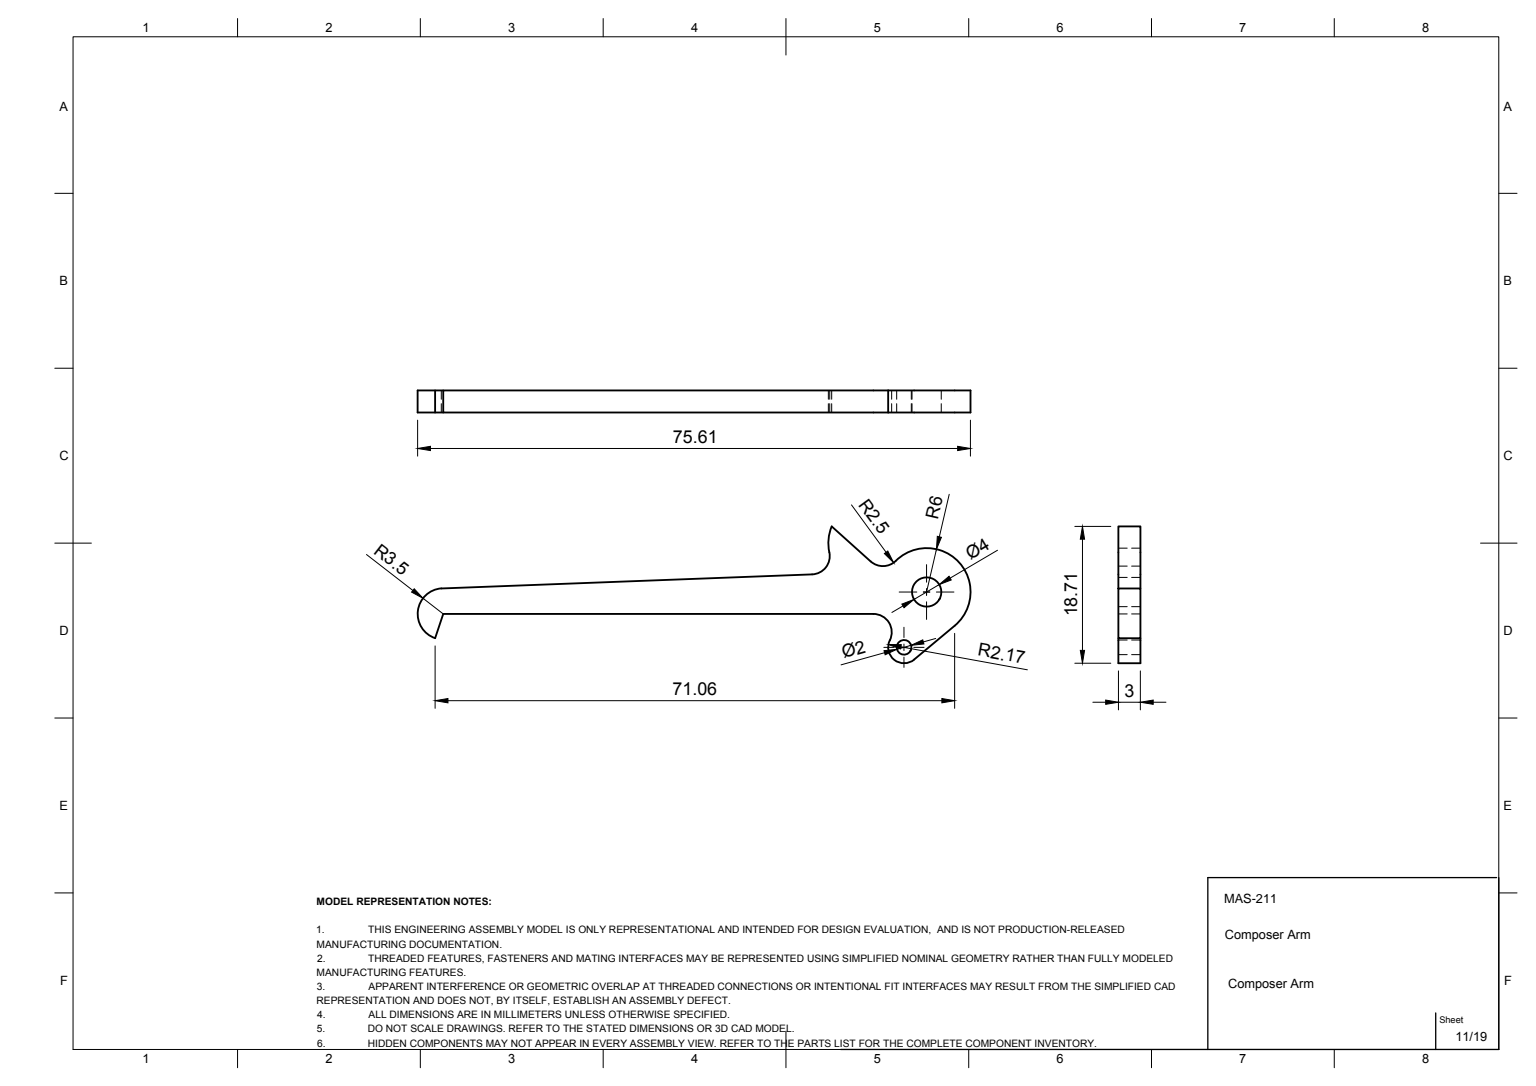
ISO-10303-21;
HEADER;
FILE_DESCRIPTION(
 (''),
 '2;1');
FILE_NAME ( 'Composer Arm.step', '2026-10-05T20:07:59+06:00', ( '' ), ( '' ), 'STEP AP214', 'Unspecified', '' );
FILE_SCHEMA (('AUTOMOTIVE_DESIGN { 1 0 10303 214 3 1 1 }'));
ENDSEC;
DATA;
#10=MECHANICAL_DESIGN_GEOMETRIC_PRESENTATION_REPRESENTATION('',(#328),#196741);
#328=STYLED_ITEM('',(#196765),#347) ;
#347=MANIFOLD_SOLID_BREP('Composer Arm',#8724) ;
#391=PLANE('',#8943) ;
#392=PLANE('',#8950) ;
#393=PLANE('',#8951) ;
#394=PLANE('',#8955) ;
#395=PLANE('',#8962) ;
#396=PLANE('',#8966) ;
#397=PLANE('',#8969) ;
#586=FACE_BOUND('',#1532,.T.) ;
#587=FACE_BOUND('',#1533,.T.) ;
#588=FACE_BOUND('',#1535,.T.) ;
#589=FACE_BOUND('',#1536,.T.) ;
#689=CIRCLE('',#8941,6.00000000000002) ;
#690=CIRCLE('',#8942,6.00000000000002) ;
#691=CIRCLE('',#8945,2.1716132700891) ;
#692=CIRCLE('',#8946,2.1716132700891) ;
#693=CIRCLE('',#8948,2.50000000000001) ;
#694=CIRCLE('',#8949,2.50000000000001) ;
#695=CIRCLE('',#8953,3.49999999999995) ;
#696=CIRCLE('',#8954,3.49999999999995) ;
#697=CIRCLE('',#8957,2.50000000000018) ;
#698=CIRCLE('',#8958,2.50000000000018) ;
#699=CIRCLE('',#8960,5.99999999999934) ;
#700=CIRCLE('',#8961,5.99999999999934) ;
#701=CIRCLE('',#8964,2.49999999999992) ;
#702=CIRCLE('',#8965,2.49999999999992) ;
#703=CIRCLE('',#8967,0.999999999999994) ;
#704=CIRCLE('',#8968,2.00000000000002) ;
#705=CIRCLE('',#8970,0.999999999999994) ;
#706=CIRCLE('',#8971,2.00000000000002) ;
#1014=FACE_OUTER_BOUND('',#1519,.T.) ;
#1015=FACE_OUTER_BOUND('',#1520,.T.) ;
#1016=FACE_OUTER_BOUND('',#1521,.T.) ;
#1017=FACE_OUTER_BOUND('',#1522,.T.) ;
#1018=FACE_OUTER_BOUND('',#1523,.T.) ;
#1019=FACE_OUTER_BOUND('',#1524,.T.) ;
#1020=FACE_OUTER_BOUND('',#1525,.T.) ;
#1021=FACE_OUTER_BOUND('',#1526,.T.) ;
#1022=FACE_OUTER_BOUND('',#1527,.T.) ;
#1023=FACE_OUTER_BOUND('',#1528,.T.) ;
#1024=FACE_OUTER_BOUND('',#1529,.T.) ;
#1025=FACE_OUTER_BOUND('',#1530,.T.) ;
#1026=FACE_OUTER_BOUND('',#1531,.T.) ;
#1027=FACE_OUTER_BOUND('',#1534,.T.) ;
#1028=FACE_OUTER_BOUND('',#1537,.T.) ;
#1029=FACE_OUTER_BOUND('',#1538,.T.) ;
#1519=EDGE_LOOP('',(#6364,#6365,#6366,#6367)) ;
#1520=EDGE_LOOP('',(#6368,#6369,#6370,#6371)) ;
#1521=EDGE_LOOP('',(#6372,#6373,#6374,#6375)) ;
#1522=EDGE_LOOP('',(#6376,#6377,#6378,#6379)) ;
#1523=EDGE_LOOP('',(#6380,#6381,#6382,#6383)) ;
#1524=EDGE_LOOP('',(#6384,#6385,#6386,#6387)) ;
#1525=EDGE_LOOP('',(#6388,#6389,#6390,#6391)) ;
#1526=EDGE_LOOP('',(#6392,#6393,#6394,#6395)) ;
#1527=EDGE_LOOP('',(#6396,#6397,#6398,#6399)) ;
#1528=EDGE_LOOP('',(#6400,#6401,#6402,#6403)) ;
#1529=EDGE_LOOP('',(#6404,#6405,#6406,#6407)) ;
#1530=EDGE_LOOP('',(#6408,#6409,#6410,#6411)) ;
#1531=EDGE_LOOP('',(#6412,#6413,#6414,#6415,#6416,#6417,#6418,#6419,#6420,
#6421,#6422,#6423)) ;
#1532=EDGE_LOOP('',(#6424)) ;
#1533=EDGE_LOOP('',(#6425)) ;
#1534=EDGE_LOOP('',(#6426,#6427,#6428,#6429,#6430,#6431,#6432,#6433,#6434,
#6435,#6436,#6437)) ;
#1535=EDGE_LOOP('',(#6438)) ;
#1536=EDGE_LOOP('',(#6439)) ;
#1537=EDGE_LOOP('',(#6440,#6441,#6442,#6443)) ;
#1538=EDGE_LOOP('',(#6444,#6445,#6446,#6447)) ;
#2010=LINE('',#113918,#2713) ;
#2011=LINE('',#113921,#2714) ;
#2012=LINE('',#113924,#2715) ;
#2013=LINE('',#113926,#2716) ;
#2014=LINE('',#113927,#2717) ;
#2015=LINE('',#113932,#2718) ;
#2016=LINE('',#113938,#2719) ;
#2017=LINE('',#113942,#2720) ;
#2018=LINE('',#113944,#2721) ;
#2019=LINE('',#113945,#2722) ;
#2020=LINE('',#113948,#2723) ;
#2021=LINE('',#113950,#2724) ;
#2022=LINE('',#113951,#2725) ;
#2023=LINE('',#113956,#2726) ;
#2024=LINE('',#113960,#2727) ;
#2025=LINE('',#113962,#2728) ;
#2026=LINE('',#113963,#2729) ;
#2027=LINE('',#113968,#2730) ;
#2028=LINE('',#113974,#2731) ;
#2029=LINE('',#113978,#2732) ;
#2030=LINE('',#113980,#2733) ;
#2031=LINE('',#113981,#2734) ;
#2032=LINE('',#113996,#2735) ;
#2033=LINE('',#113998,#2736) ;
#2713=VECTOR('',#9994,10.) ;
#2714=VECTOR('',#9997,10.) ;
#2715=VECTOR('',#10000,10.) ;
#2716=VECTOR('',#10001,10.) ;
#2717=VECTOR('',#10002,10.) ;
#2718=VECTOR('',#10007,10.) ;
#2719=VECTOR('',#10014,10.) ;
#2720=VECTOR('',#10019,10.) ;
#2721=VECTOR('',#10020,10.) ;
#2722=VECTOR('',#10021,10.) ;
#2723=VECTOR('',#10024,10.) ;
#2724=VECTOR('',#10025,10.) ;
#2725=VECTOR('',#10026,10.) ;
#2726=VECTOR('',#10031,10.) ;
#2727=VECTOR('',#10036,10.) ;
#2728=VECTOR('',#10037,10.) ;
#2729=VECTOR('',#10038,10.) ;
#2730=VECTOR('',#10043,10.) ;
#2731=VECTOR('',#10050,10.) ;
#2732=VECTOR('',#10055,10.) ;
#2733=VECTOR('',#10056,10.) ;
#2734=VECTOR('',#10057,10.) ;
#2735=VECTOR('',#10078,1.00000000000007) ;
#2736=VECTOR('',#10081,2.00000000000001) ;
#3708=VERTEX_POINT('',#113914) ;
#3709=VERTEX_POINT('',#113915) ;
#3710=VERTEX_POINT('',#113917) ;
#3711=VERTEX_POINT('',#113919) ;
#3712=VERTEX_POINT('',#113923) ;
#3713=VERTEX_POINT('',#113925) ;
#3714=VERTEX_POINT('',#113929) ;
#3715=VERTEX_POINT('',#113931) ;
#3716=VERTEX_POINT('',#113935) ;
#3717=VERTEX_POINT('',#113937) ;
#3718=VERTEX_POINT('',#113941) ;
#3719=VERTEX_POINT('',#113943) ;
#3720=VERTEX_POINT('',#113947) ;
#3721=VERTEX_POINT('',#113949) ;
#3722=VERTEX_POINT('',#113953) ;
#3723=VERTEX_POINT('',#113955) ;
#3724=VERTEX_POINT('',#113959) ;
#3725=VERTEX_POINT('',#113961) ;
#3726=VERTEX_POINT('',#113965) ;
#3727=VERTEX_POINT('',#113967) ;
#3728=VERTEX_POINT('',#113971) ;
#3729=VERTEX_POINT('',#113973) ;
#3730=VERTEX_POINT('',#113977) ;
#3731=VERTEX_POINT('',#113979) ;
#3732=VERTEX_POINT('',#113986) ;
#3733=VERTEX_POINT('',#113988) ;
#3734=VERTEX_POINT('',#113991) ;
#3735=VERTEX_POINT('',#113993) ;
#4690=EDGE_CURVE('',#3708,#3709,#689,.T.) ;
#4691=EDGE_CURVE('',#3709,#3710,#2010,.T.) ;
#4692=EDGE_CURVE('',#3711,#3710,#690,.T.) ;
#4693=EDGE_CURVE('',#3708,#3711,#2011,.T.) ;
#4694=EDGE_CURVE('',#3709,#3712,#2012,.T.) ;
#4695=EDGE_CURVE('',#3712,#3713,#2013,.T.) ;
#4696=EDGE_CURVE('',#3710,#3713,#2014,.T.) ;
#4697=EDGE_CURVE('',#3712,#3714,#691,.T.) ;
#4698=EDGE_CURVE('',#3714,#3715,#2015,.T.) ;
#4699=EDGE_CURVE('',#3713,#3715,#692,.T.) ;
#4700=EDGE_CURVE('',#3714,#3716,#693,.T.) ;
#4701=EDGE_CURVE('',#3716,#3717,#2016,.T.) ;
#4702=EDGE_CURVE('',#3715,#3717,#694,.T.) ;
#4703=EDGE_CURVE('',#3716,#3718,#2017,.T.) ;
#4704=EDGE_CURVE('',#3718,#3719,#2018,.T.) ;
#4705=EDGE_CURVE('',#3717,#3719,#2019,.T.) ;
#4706=EDGE_CURVE('',#3718,#3720,#2020,.T.) ;
#4707=EDGE_CURVE('',#3720,#3721,#2021,.T.) ;
#4708=EDGE_CURVE('',#3719,#3721,#2022,.T.) ;
#4709=EDGE_CURVE('',#3720,#3722,#695,.T.) ;
#4710=EDGE_CURVE('',#3722,#3723,#2023,.T.) ;
#4711=EDGE_CURVE('',#3721,#3723,#696,.T.) ;
#4712=EDGE_CURVE('',#3722,#3724,#2024,.T.) ;
#4713=EDGE_CURVE('',#3724,#3725,#2025,.T.) ;
#4714=EDGE_CURVE('',#3723,#3725,#2026,.T.) ;
#4715=EDGE_CURVE('',#3724,#3726,#697,.T.) ;
#4716=EDGE_CURVE('',#3726,#3727,#2027,.T.) ;
#4717=EDGE_CURVE('',#3725,#3727,#698,.T.) ;
#4718=EDGE_CURVE('',#3726,#3728,#699,.T.) ;
#4719=EDGE_CURVE('',#3728,#3729,#2028,.T.) ;
#4720=EDGE_CURVE('',#3727,#3729,#700,.T.) ;
#4721=EDGE_CURVE('',#3728,#3730,#2029,.T.) ;
#4722=EDGE_CURVE('',#3730,#3731,#2030,.T.) ;
#4723=EDGE_CURVE('',#3729,#3731,#2031,.T.) ;
#4724=EDGE_CURVE('',#3730,#3708,#701,.T.) ;
#4725=EDGE_CURVE('',#3731,#3711,#702,.T.) ;
#4726=EDGE_CURVE('',#3732,#3732,#703,.T.) ;
#4727=EDGE_CURVE('',#3733,#3733,#704,.T.) ;
#4728=EDGE_CURVE('',#3734,#3734,#705,.T.) ;
#4729=EDGE_CURVE('',#3735,#3735,#706,.T.) ;
#4730=EDGE_CURVE('',#3734,#3732,#2032,.T.) ;
#4731=EDGE_CURVE('',#3733,#3735,#2033,.T.) ;
#6364=ORIENTED_EDGE('',*,*,#4690,.T.) ;
#6365=ORIENTED_EDGE('',*,*,#4691,.T.) ;
#6366=ORIENTED_EDGE('',*,*,#4692,.F.) ;
#6367=ORIENTED_EDGE('',*,*,#4693,.F.) ;
#6368=ORIENTED_EDGE('',*,*,#4694,.T.) ;
#6369=ORIENTED_EDGE('',*,*,#4695,.T.) ;
#6370=ORIENTED_EDGE('',*,*,#4696,.F.) ;
#6371=ORIENTED_EDGE('',*,*,#4691,.F.) ;
#6372=ORIENTED_EDGE('',*,*,#4697,.T.) ;
#6373=ORIENTED_EDGE('',*,*,#4698,.T.) ;
#6374=ORIENTED_EDGE('',*,*,#4699,.F.) ;
#6375=ORIENTED_EDGE('',*,*,#4695,.F.) ;
#6376=ORIENTED_EDGE('',*,*,#4700,.T.) ;
#6377=ORIENTED_EDGE('',*,*,#4701,.T.) ;
#6378=ORIENTED_EDGE('',*,*,#4702,.F.) ;
#6379=ORIENTED_EDGE('',*,*,#4698,.F.) ;
#6380=ORIENTED_EDGE('',*,*,#4703,.T.) ;
#6381=ORIENTED_EDGE('',*,*,#4704,.T.) ;
#6382=ORIENTED_EDGE('',*,*,#4705,.F.) ;
#6383=ORIENTED_EDGE('',*,*,#4701,.F.) ;
#6384=ORIENTED_EDGE('',*,*,#4706,.T.) ;
#6385=ORIENTED_EDGE('',*,*,#4707,.T.) ;
#6386=ORIENTED_EDGE('',*,*,#4708,.F.) ;
#6387=ORIENTED_EDGE('',*,*,#4704,.F.) ;
#6388=ORIENTED_EDGE('',*,*,#4709,.T.) ;
#6389=ORIENTED_EDGE('',*,*,#4710,.T.) ;
#6390=ORIENTED_EDGE('',*,*,#4711,.F.) ;
#6391=ORIENTED_EDGE('',*,*,#4707,.F.) ;
#6392=ORIENTED_EDGE('',*,*,#4712,.T.) ;
#6393=ORIENTED_EDGE('',*,*,#4713,.T.) ;
#6394=ORIENTED_EDGE('',*,*,#4714,.F.) ;
#6395=ORIENTED_EDGE('',*,*,#4710,.F.) ;
#6396=ORIENTED_EDGE('',*,*,#4715,.T.) ;
#6397=ORIENTED_EDGE('',*,*,#4716,.T.) ;
#6398=ORIENTED_EDGE('',*,*,#4717,.F.) ;
#6399=ORIENTED_EDGE('',*,*,#4713,.F.) ;
#6400=ORIENTED_EDGE('',*,*,#4718,.T.) ;
#6401=ORIENTED_EDGE('',*,*,#4719,.T.) ;
#6402=ORIENTED_EDGE('',*,*,#4720,.F.) ;
#6403=ORIENTED_EDGE('',*,*,#4716,.F.) ;
#6404=ORIENTED_EDGE('',*,*,#4721,.T.) ;
#6405=ORIENTED_EDGE('',*,*,#4722,.T.) ;
#6406=ORIENTED_EDGE('',*,*,#4723,.F.) ;
#6407=ORIENTED_EDGE('',*,*,#4719,.F.) ;
#6408=ORIENTED_EDGE('',*,*,#4724,.T.) ;
#6409=ORIENTED_EDGE('',*,*,#4693,.T.) ;
#6410=ORIENTED_EDGE('',*,*,#4725,.F.) ;
#6411=ORIENTED_EDGE('',*,*,#4722,.F.) ;
#6412=ORIENTED_EDGE('',*,*,#4724,.F.) ;
#6413=ORIENTED_EDGE('',*,*,#4721,.F.) ;
#6414=ORIENTED_EDGE('',*,*,#4718,.F.) ;
#6415=ORIENTED_EDGE('',*,*,#4715,.F.) ;
#6416=ORIENTED_EDGE('',*,*,#4712,.F.) ;
#6417=ORIENTED_EDGE('',*,*,#4709,.F.) ;
#6418=ORIENTED_EDGE('',*,*,#4706,.F.) ;
#6419=ORIENTED_EDGE('',*,*,#4703,.F.) ;
#6420=ORIENTED_EDGE('',*,*,#4700,.F.) ;
#6421=ORIENTED_EDGE('',*,*,#4697,.F.) ;
#6422=ORIENTED_EDGE('',*,*,#4694,.F.) ;
#6423=ORIENTED_EDGE('',*,*,#4690,.F.) ;
#6424=ORIENTED_EDGE('',*,*,#4726,.F.) ;
#6425=ORIENTED_EDGE('',*,*,#4727,.F.) ;
#6426=ORIENTED_EDGE('',*,*,#4692,.T.) ;
#6427=ORIENTED_EDGE('',*,*,#4696,.T.) ;
#6428=ORIENTED_EDGE('',*,*,#4699,.T.) ;
#6429=ORIENTED_EDGE('',*,*,#4702,.T.) ;
#6430=ORIENTED_EDGE('',*,*,#4705,.T.) ;
#6431=ORIENTED_EDGE('',*,*,#4708,.T.) ;
#6432=ORIENTED_EDGE('',*,*,#4711,.T.) ;
#6433=ORIENTED_EDGE('',*,*,#4714,.T.) ;
#6434=ORIENTED_EDGE('',*,*,#4717,.T.) ;
#6435=ORIENTED_EDGE('',*,*,#4720,.T.) ;
#6436=ORIENTED_EDGE('',*,*,#4723,.T.) ;
#6437=ORIENTED_EDGE('',*,*,#4725,.T.) ;
#6438=ORIENTED_EDGE('',*,*,#4728,.T.) ;
#6439=ORIENTED_EDGE('',*,*,#4729,.T.) ;
#6440=ORIENTED_EDGE('',*,*,#4728,.F.) ;
#6441=ORIENTED_EDGE('',*,*,#4730,.T.) ;
#6442=ORIENTED_EDGE('',*,*,#4726,.T.) ;
#6443=ORIENTED_EDGE('',*,*,#4730,.F.) ;
#6444=ORIENTED_EDGE('',*,*,#4727,.T.) ;
#6445=ORIENTED_EDGE('',*,*,#4731,.T.) ;
#6446=ORIENTED_EDGE('',*,*,#4729,.F.) ;
#6447=ORIENTED_EDGE('',*,*,#4731,.F.) ;
#8185=CYLINDRICAL_SURFACE('',#8940,5.99999999999987) ;
#8186=CYLINDRICAL_SURFACE('',#8944,2.17161327008925) ;
#8187=CYLINDRICAL_SURFACE('',#8947,2.49999999999937) ;
#8188=CYLINDRICAL_SURFACE('',#8952,3.50000000000016) ;
#8189=CYLINDRICAL_SURFACE('',#8956,2.50000000000004) ;
#8190=CYLINDRICAL_SURFACE('',#8959,5.99999999999939) ;
#8191=CYLINDRICAL_SURFACE('',#8963,2.49999999999973) ;
#8192=CYLINDRICAL_SURFACE('',#8972,1.00000000000007) ;
#8193=CYLINDRICAL_SURFACE('',#8973,2.00000000000001) ;
#8397=ADVANCED_FACE('',(#1014),#8185,.T.) ;
#8398=ADVANCED_FACE('',(#1015),#391,.T.) ;
#8399=ADVANCED_FACE('',(#1016),#8186,.T.) ;
#8400=ADVANCED_FACE('',(#1017),#8187,.F.) ;
#8401=ADVANCED_FACE('',(#1018),#392,.T.) ;
#8402=ADVANCED_FACE('',(#1019),#393,.T.) ;
#8403=ADVANCED_FACE('',(#1020),#8188,.T.) ;
#8404=ADVANCED_FACE('',(#1021),#394,.T.) ;
#8405=ADVANCED_FACE('',(#1022),#8189,.F.) ;
#8406=ADVANCED_FACE('',(#1023),#8190,.T.) ;
#8407=ADVANCED_FACE('',(#1024),#395,.T.) ;
#8408=ADVANCED_FACE('',(#1025),#8191,.F.) ;
#8409=ADVANCED_FACE('',(#1026,#586,#587),#396,.T.) ;
#8410=ADVANCED_FACE('',(#1027,#588,#589),#397,.T.) ;
#8411=ADVANCED_FACE('',(#1028),#8192,.F.) ;
#8412=ADVANCED_FACE('',(#1029),#8193,.F.) ;
#8724=CLOSED_SHELL('',(#8397,#8398,#8399,#8400,#8401,#8402,#8403,#8404,
#8405,#8406,#8407,#8408,#8409,#8410,#8411,#8412)) ;
#8940=AXIS2_PLACEMENT_3D('',#113913,#9990,#9991) ;
#8941=AXIS2_PLACEMENT_3D('',#113916,#9992,#9993) ;
#8942=AXIS2_PLACEMENT_3D('',#113920,#9995,#9996) ;
#8943=AXIS2_PLACEMENT_3D('',#113922,#9998,#9999) ;
#8944=AXIS2_PLACEMENT_3D('',#113928,#10003,#10004) ;
#8945=AXIS2_PLACEMENT_3D('',#113930,#10005,#10006) ;
#8946=AXIS2_PLACEMENT_3D('',#113933,#10008,#10009) ;
#8947=AXIS2_PLACEMENT_3D('',#113934,#10010,#10011) ;
#8948=AXIS2_PLACEMENT_3D('',#113936,#10012,#10013) ;
#8949=AXIS2_PLACEMENT_3D('',#113939,#10015,#10016) ;
#8950=AXIS2_PLACEMENT_3D('',#113940,#10017,#10018) ;
#8951=AXIS2_PLACEMENT_3D('',#113946,#10022,#10023) ;
#8952=AXIS2_PLACEMENT_3D('',#113952,#10027,#10028) ;
#8953=AXIS2_PLACEMENT_3D('',#113954,#10029,#10030) ;
#8954=AXIS2_PLACEMENT_3D('',#113957,#10032,#10033) ;
#8955=AXIS2_PLACEMENT_3D('',#113958,#10034,#10035) ;
#8956=AXIS2_PLACEMENT_3D('',#113964,#10039,#10040) ;
#8957=AXIS2_PLACEMENT_3D('',#113966,#10041,#10042) ;
#8958=AXIS2_PLACEMENT_3D('',#113969,#10044,#10045) ;
#8959=AXIS2_PLACEMENT_3D('',#113970,#10046,#10047) ;
#8960=AXIS2_PLACEMENT_3D('',#113972,#10048,#10049) ;
#8961=AXIS2_PLACEMENT_3D('',#113975,#10051,#10052) ;
#8962=AXIS2_PLACEMENT_3D('',#113976,#10053,#10054) ;
#8963=AXIS2_PLACEMENT_3D('',#113982,#10058,#10059) ;
#8964=AXIS2_PLACEMENT_3D('',#113983,#10060,#10061) ;
#8965=AXIS2_PLACEMENT_3D('',#113984,#10062,#10063) ;
#8966=AXIS2_PLACEMENT_3D('',#113985,#10064,#10065) ;
#8967=AXIS2_PLACEMENT_3D('',#113987,#10066,#10067) ;
#8968=AXIS2_PLACEMENT_3D('',#113989,#10068,#10069) ;
#8969=AXIS2_PLACEMENT_3D('',#113990,#10070,#10071) ;
#8970=AXIS2_PLACEMENT_3D('',#113992,#10072,#10073) ;
#8971=AXIS2_PLACEMENT_3D('',#113994,#10074,#10075) ;
#8972=AXIS2_PLACEMENT_3D('',#113995,#10076,#10077) ;
#8973=AXIS2_PLACEMENT_3D('',#113997,#10079,#10080) ;
#9990=DIRECTION('center_axis',(0.,1.,0.)) ;
#9991=DIRECTION('ref_axis',(-0.323408449520454,0.,0.946259464829164)) ;
#9992=DIRECTION('center_axis',(0.,-1.,0.)) ;
#9993=DIRECTION('ref_axis',(-0.931688169129028,0.,-0.36325907491073)) ;
#9994=DIRECTION('',(0.,-1.,0.)) ;
#9995=DIRECTION('center_axis',(0.,-1.,0.)) ;
#9996=DIRECTION('ref_axis',(-0.931688169129028,0.,-0.36325907491073)) ;
#9997=DIRECTION('',(0.,-1.,0.)) ;
#9998=DIRECTION('center_axis',(-0.931688169129027,0.,-0.363259074910734)) ;
#9999=DIRECTION('ref_axis',(-0.363259074910734,0.,0.931688169129026)) ;
#10000=DIRECTION('',(0.363259074910734,0.,-0.931688169129027)) ;
#10001=DIRECTION('',(0.,-1.,0.)) ;
#10002=DIRECTION('',(0.363259074910734,0.,-0.931688169129027)) ;
#10003=DIRECTION('center_axis',(0.,1.,0.)) ;
#10004=DIRECTION('ref_axis',(0.162186831709887,0.,-0.986760067909068)) ;
#10005=DIRECTION('center_axis',(0.,-1.,0.)) ;
#10006=DIRECTION('ref_axis',(0.998944452320448,0.,-0.0459345314355166)) ;
#10007=DIRECTION('',(0.,-1.,0.)) ;
#10008=DIRECTION('center_axis',(0.,-1.,0.)) ;
#10009=DIRECTION('ref_axis',(0.998944452320448,0.,-0.0459345314355166)) ;
#10010=DIRECTION('center_axis',(0.,-1.,0.)) ;
#10011=DIRECTION('ref_axis',(-0.488673380771942,0.,0.872466805629257)) ;
#10012=DIRECTION('center_axis',(0.,1.,0.)) ;
#10013=DIRECTION('ref_axis',(0.48267674456582,0.,0.875798584296265)) ;
#10014=DIRECTION('',(0.,-1.,0.)) ;
#10015=DIRECTION('center_axis',(0.,1.,0.)) ;
#10016=DIRECTION('ref_axis',(0.48267674456582,0.,0.875798584296265)) ;
#10017=DIRECTION('center_axis',(-0.482676744565949,0.,-0.875798584296194)) ;
#10018=DIRECTION('ref_axis',(-0.875798584296194,0.,0.482676744565949)) ;
#10019=DIRECTION('',(0.875798584296194,0.,-0.482676744565949)) ;
#10020=DIRECTION('',(0.,-1.,0.)) ;
#10021=DIRECTION('',(0.875798584296194,0.,-0.482676744565949)) ;
#10022=DIRECTION('center_axis',(-0.983502142252922,0.,0.180896479191588)) ;
#10023=DIRECTION('ref_axis',(0.180896479191588,0.,0.983502142252922)) ;
#10024=DIRECTION('',(-0.180896479191588,0.,-0.983502142252922)) ;
#10025=DIRECTION('',(0.,-1.,0.)) ;
#10026=DIRECTION('',(-0.180896479191588,0.,-0.983502142252922)) ;
#10027=DIRECTION('center_axis',(0.,1.,0.)) ;
#10028=DIRECTION('ref_axis',(0.928762380268974,0.,-0.370675654713267)) ;
#10029=DIRECTION('center_axis',(0.,-1.,0.)) ;
#10030=DIRECTION('ref_axis',(0.545993817711977,0.,0.837789204406634)) ;
#10031=DIRECTION('',(0.,-1.,0.)) ;
#10032=DIRECTION('center_axis',(0.,-1.,0.)) ;
#10033=DIRECTION('ref_axis',(0.545993817711977,0.,0.837789204406634)) ;
#10034=DIRECTION('center_axis',(0.515454087003814,0.,0.856917197978349)) ;
#10035=DIRECTION('ref_axis',(0.856917197978349,0.,-0.515454087003814)) ;
#10036=DIRECTION('',(-0.856917197978349,0.,0.515454087003814)) ;
#10037=DIRECTION('',(0.,-1.,0.)) ;
#10038=DIRECTION('',(-0.856917197978349,0.,0.515454087003814)) ;
#10039=DIRECTION('center_axis',(0.,-1.,0.)) ;
#10040=DIRECTION('ref_axis',(-0.98759867396716,0.,-0.156999551522628)) ;
#10041=DIRECTION('center_axis',(0.,1.,0.)) ;
#10042=DIRECTION('ref_axis',(-0.755777768077742,0.,0.654828195238588)) ;
#10043=DIRECTION('',(0.,-1.,0.)) ;
#10044=DIRECTION('center_axis',(0.,1.,0.)) ;
#10045=DIRECTION('ref_axis',(-0.755777768077742,0.,0.654828195238588)) ;
#10046=DIRECTION('center_axis',(0.,1.,0.)) ;
#10047=DIRECTION('ref_axis',(0.915970102946441,0.,-0.401246520867516)) ;
#10048=DIRECTION('center_axis',(7.3591138693603E-18,-1.,-3.22370656776922E-18)) ;
#10049=DIRECTION('ref_axis',(0.993756958760637,7.58941520739936E-18,-0.111566603044145)) ;
#10050=DIRECTION('',(0.,-1.,0.)) ;
#10051=DIRECTION('center_axis',(3.76786630111247E-15,-1.,-1.65053776269784E-15)) ;
#10052=DIRECTION('ref_axis',(0.993756958760637,3.88578058618847E-15,-0.111566603044145)) ;
#10053=DIRECTION('center_axis',(-0.226066317498263,0.,0.974111913536004)) ;
#10054=DIRECTION('ref_axis',(0.974111913536004,0.,0.226066317498263)) ;
#10055=DIRECTION('',(-0.974111913536004,0.,-0.226066317498263)) ;
#10056=DIRECTION('',(0.,-1.,0.)) ;
#10057=DIRECTION('',(-0.974111913536004,0.,-0.226066317498263)) ;
#10058=DIRECTION('center_axis',(0.,-1.,0.)) ;
#10059=DIRECTION('ref_axis',(-0.503747852925287,0.,-0.863850739811667)) ;
#10060=DIRECTION('center_axis',(0.,1.,0.)) ;
#10061=DIRECTION('ref_axis',(-0.959127119717865,0.,-0.28297556117395)) ;
#10062=DIRECTION('center_axis',(4.10636256070708E-16,1.,7.04178551908964E-16)) ;
#10063=DIRECTION('ref_axis',(-0.959127119717865,6.66133814775114E-16,-0.28297556117395)) ;
#10064=DIRECTION('center_axis',(0.,1.,0.)) ;
#10065=DIRECTION('ref_axis',(0.,0.,1.)) ;
#10066=DIRECTION('center_axis',(-1.1978755459731E-19,1.,3.59810729949512E-18)) ;
#10067=DIRECTION('ref_axis',(0.875530529285933,-2.16840434497102E-18,0.48316280101876)) ;
#10068=DIRECTION('center_axis',(-6.93236427336665E-16,1.,-9.96444582969986E-17)) ;
#10069=DIRECTION('ref_axis',(-0.948327476740892,-6.2558465352413E-16,0.317293234813244)) ;
#10070=DIRECTION('center_axis',(0.,-1.,0.)) ;
#10071=DIRECTION('ref_axis',(0.,0.,-1.)) ;
#10072=DIRECTION('center_axis',(2.78998493207323E-16,1.,5.4878418411934E-17)) ;
#10073=DIRECTION('ref_axis',(0.875530529285933,0.,0.48316280101876)) ;
#10074=DIRECTION('center_axis',(1.14634110235167E-16,1.,-8.40950104074492E-17)) ;
#10075=DIRECTION('ref_axis',(-0.948327476740892,0.,0.317293234813244)) ;
#10076=DIRECTION('center_axis',(0.,-1.,0.)) ;
#10077=DIRECTION('ref_axis',(0.993299589837987,0.,-0.115567836475751)) ;
#10078=DIRECTION('',(0.,1.,0.)) ;
#10079=DIRECTION('center_axis',(0.,1.,0.)) ;
#10080=DIRECTION('ref_axis',(-0.587391769794674,0.,0.809302729995075)) ;
#10081=DIRECTION('',(0.,-1.,0.)) ;
#113913=CARTESIAN_POINT('Origin',(-28.8703041205687,-0.0122621421566816,
120.173187866852)) ;
#113914=CARTESIAN_POINT('',(-23.1155414022614,-0.0122621421566816,121.871041233896)) ;
#113915=CARTESIAN_POINT('',(-34.4604331353428,-0.0122621421566816,117.993633417388)) ;
#113916=CARTESIAN_POINT('Origin',(-28.8703041205686,-0.0122621421566816,
120.173187866852)) ;
#113917=CARTESIAN_POINT('',(-34.4604331353428,-3.01226214215668,117.993633417388)) ;
#113918=CARTESIAN_POINT('',(-34.4604331353428,-0.0122621421566816,117.993633417388)) ;
#113919=CARTESIAN_POINT('',(-23.1155414022614,-3.01226214215668,121.871041233896)) ;
#113920=CARTESIAN_POINT('Origin',(-28.8703041205686,-3.01226214215668,120.173187866852)) ;
#113921=CARTESIAN_POINT('',(-23.1155414022614,-0.0122621421566816,121.871041233896)) ;
#113922=CARTESIAN_POINT('Origin',(-33.1491896568585,-0.0122621421566816,
114.630551473595)) ;
#113923=CARTESIAN_POINT('',(-31.8379461783745,-0.0122621421566816,111.267469529802)) ;
#113924=CARTESIAN_POINT('',(-34.4604331353428,-0.0122621421566816,117.993633417388)) ;
#113925=CARTESIAN_POINT('',(-31.8379461783745,-3.01226214215668,111.267469529802)) ;
#113926=CARTESIAN_POINT('',(-31.8379461783745,-0.0122621421566816,111.267469529802)) ;
#113927=CARTESIAN_POINT('',(-34.4604331353428,-3.01226214215668,117.993633417388)) ;
#113928=CARTESIAN_POINT('Origin',(-29.8146797867087,-0.0122621421566816,
112.056327757358)) ;
#113929=CARTESIAN_POINT('',(-27.6453587579679,-0.0122621421566816,111.956575719337)) ;
#113930=CARTESIAN_POINT('Origin',(-29.8146797867088,-0.0122621421566816,
112.056327757358)) ;
#113931=CARTESIAN_POINT('',(-27.6453587579679,-3.01226214215668,111.956575719337)) ;
#113932=CARTESIAN_POINT('',(-27.6453587579679,-0.0122621421566816,111.956575719337)) ;
#113933=CARTESIAN_POINT('Origin',(-29.8146797867088,-3.01226214215668,112.056327757358)) ;
#113934=CARTESIAN_POINT('Origin',(-25.1479976271673,-0.0122621421566816,
111.841739390749)) ;
#113935=CARTESIAN_POINT('',(-23.9413057657522,-0.0122621421566816,114.031235851489)) ;
#113936=CARTESIAN_POINT('Origin',(-25.1479976271667,-0.0122621421566816,
111.841739390748)) ;
#113937=CARTESIAN_POINT('',(-23.9413057657522,-3.01226214215668,114.031235851489)) ;
#113938=CARTESIAN_POINT('',(-23.9413057657522,-0.0122621421566816,114.031235851489)) ;
#113939=CARTESIAN_POINT('Origin',(-25.1479976271667,-3.01226214215668,111.841739390748)) ;
#113940=CARTESIAN_POINT('Origin',(1.81795236235752,-0.0122621421566816,
99.834598543949)) ;
#113941=CARTESIAN_POINT('',(27.5772104904673,-0.0122621421566816,85.6379612364092)) ;
#113942=CARTESIAN_POINT('',(-23.9413057657522,-0.0122621421566816,114.031235851489)) ;
#113943=CARTESIAN_POINT('',(27.5772104904673,-3.01226214215668,85.6379612364092)) ;
#113944=CARTESIAN_POINT('',(27.5772104904673,-0.0122621421566816,85.6379612364092)) ;
#113945=CARTESIAN_POINT('',(-23.9413057657522,-3.01226214215668,114.031235851489)) ;
#113946=CARTESIAN_POINT('Origin',(27.2606416518821,-0.0122621421566816,
83.9168324874666)) ;
#113947=CARTESIAN_POINT('',(26.9440728132968,-0.0122621421566816,82.1957037385239)) ;
#113948=CARTESIAN_POINT('',(27.5772104904673,-0.0122621421566816,85.6379612364092)) ;
#113949=CARTESIAN_POINT('',(26.9440728132968,-3.01226214215668,82.1957037385239)) ;
#113950=CARTESIAN_POINT('',(26.9440728132968,-0.0122621421566816,82.1957037385239)) ;
#113951=CARTESIAN_POINT('',(27.5772104904673,-3.01226214215668,85.6379612364092)) ;
#113952=CARTESIAN_POINT('Origin',(27.5772104904672,-0.0122621421566816,
85.6379612364093)) ;
#113953=CARTESIAN_POINT('',(29.4881888524592,-0.0122621421566816,88.5702234518323)) ;
#113954=CARTESIAN_POINT('Origin',(27.5772104904673,-0.0122621421566816,
85.6379612364091)) ;
#113955=CARTESIAN_POINT('',(29.4881888524592,-3.01226214215668,88.5702234518323)) ;
#113956=CARTESIAN_POINT('',(29.4881888524592,-0.0122621421566816,88.5702234518323)) ;
#113957=CARTESIAN_POINT('Origin',(27.5772104904673,-3.01226214215668,85.6379612364091)) ;
#113958=CARTESIAN_POINT('Origin',(7.74723983920157,-0.0122621421566816,
101.647870919597)) ;
#113959=CARTESIAN_POINT('',(-13.9937091740561,-0.0122621421566816,114.725518387361)) ;
#113960=CARTESIAN_POINT('',(29.4881888524592,-0.0122621421566816,88.5702234518323)) ;
#113961=CARTESIAN_POINT('',(-13.9937091740561,-3.01226214215668,114.725518387361)) ;
#113962=CARTESIAN_POINT('',(-13.9937091740561,-0.0122621421566816,114.725518387361)) ;
#113963=CARTESIAN_POINT('',(29.4881888524592,-3.01226214215668,88.5702234518323)) ;
#113964=CARTESIAN_POINT('Origin',(-12.7050739565465,-0.0122621421566816,
116.867811382307)) ;
#113965=CARTESIAN_POINT('',(-14.5945183767409,-0.0122621421566816,118.504881870403)) ;
#113966=CARTESIAN_POINT('Origin',(-12.7050739565464,-0.0122621421566816,
116.867811382307)) ;
#113967=CARTESIAN_POINT('',(-14.5945183767409,-3.01226214215668,118.504881870403)) ;
#113968=CARTESIAN_POINT('',(-14.5945183767409,-0.0122621421566816,118.504881870403)) ;
#113969=CARTESIAN_POINT('Origin',(-12.7050739565464,-3.01226214215668,116.867811382307)) ;
#113970=CARTESIAN_POINT('Origin',(-19.1291849852063,-0.0122621421566816,
122.433851041835)) ;
#113971=CARTESIAN_POINT('',(-13.1666432326431,-0.0122621421566816,121.76445142357)) ;
#113972=CARTESIAN_POINT('Origin',(-19.1291849852063,-0.0122621421566816,
122.433851041835)) ;
#113973=CARTESIAN_POINT('',(-13.1666432326431,-3.01226214215668,121.76445142357)) ;
#113974=CARTESIAN_POINT('',(-13.1666432326431,-0.0122621421566816,121.76445142357)) ;
#113975=CARTESIAN_POINT('Origin',(-19.1291849852063,-3.01226214215671,122.433851041835)) ;
#113976=CARTESIAN_POINT('Origin',(-16.6596005209322,-0.0122621421566816,
120.953825888281)) ;
#113977=CARTESIAN_POINT('',(-20.1525578092214,-0.0122621421566816,120.143200352991)) ;
#113978=CARTESIAN_POINT('',(-13.1666432326431,-0.0122621421566816,121.76445142357)) ;
#113979=CARTESIAN_POINT('',(-20.1525578092214,-3.01226214215668,120.143200352991)) ;
#113980=CARTESIAN_POINT('',(-20.1525578092214,-0.0122621421566816,120.143200352991)) ;
#113981=CARTESIAN_POINT('',(-13.1666432326431,-3.01226214215668,121.76445142357)) ;
#113982=CARTESIAN_POINT('Origin',(-20.7177236029669,-0.0122621421566816,
122.578480136831)) ;
#113983=CARTESIAN_POINT('Origin',(-20.7177236029668,-0.0122621421566816,
122.578480136831)) ;
#113984=CARTESIAN_POINT('Origin',(-20.7177236029668,-3.01226214215668,122.578480136831)) ;
#113985=CARTESIAN_POINT('Origin',(-23.1155414022614,-0.0122621421566816,
121.871041233896)) ;
#113986=CARTESIAN_POINT('',(-30.807979376547,-0.0122621421566815,112.171895593834)) ;
#113987=CARTESIAN_POINT('Origin',(-29.8146797867089,-0.0122621421566816,
112.056327757358)) ;
#113988=CARTESIAN_POINT('',(-27.6955205809792,-0.0122621421566782,118.554582406862)) ;
#113989=CARTESIAN_POINT('Origin',(-28.8703041205685,-0.0122621421566797,
120.173187866852)) ;
#113990=CARTESIAN_POINT('Origin',(-23.1155414022614,-3.01226214215668,121.871041233896)) ;
#113991=CARTESIAN_POINT('',(-30.807979376547,-3.01226214215668,112.171895593834)) ;
#113992=CARTESIAN_POINT('Origin',(-29.8146797867089,-3.01226214215668,112.056327757358)) ;
#113993=CARTESIAN_POINT('',(-27.6955205809792,-3.01226214215668,118.554582406862)) ;
#113994=CARTESIAN_POINT('Origin',(-28.8703041205685,-3.01226214215668,120.173187866852)) ;
#113995=CARTESIAN_POINT('Origin',(-29.814679786709,-6.99999999995041,112.056327757358)) ;
#113996=CARTESIAN_POINT('',(-30.807979376547,-6.99999999995041,112.171895593834)) ;
#113997=CARTESIAN_POINT('Origin',(-28.8703041205685,0.,120.173187866852)) ;
#113998=CARTESIAN_POINT('',(-27.6955205809792,0.,118.554582406862)) ;
#196737=UNCERTAINTY_MEASURE_WITH_UNIT(LENGTH_MEASURE(0.01),#196742,
'DISTANCE_ACCURACY_VALUE',
'Maximum model space distance between geometric entities at asserted c
onnectivities') ;
#196738=UNCERTAINTY_MEASURE_WITH_UNIT(LENGTH_MEASURE(0.01),#196742,
'DISTANCE_ACCURACY_VALUE',
'Maximum model space distance between geometric entities at asserted c
onnectivities') ;
#196740=(
GEOMETRIC_REPRESENTATION_CONTEXT(3)
GLOBAL_UNCERTAINTY_ASSIGNED_CONTEXT((#196737))
GLOBAL_UNIT_ASSIGNED_CONTEXT((#196742,#196744,#196745))
REPRESENTATION_CONTEXT('','3D')
) ;
#196741=(
GEOMETRIC_REPRESENTATION_CONTEXT(3)
GLOBAL_UNCERTAINTY_ASSIGNED_CONTEXT((#196738))
GLOBAL_UNIT_ASSIGNED_CONTEXT((#196742,#196744,#196745))
REPRESENTATION_CONTEXT('','3D')
) ;
#196742=(
LENGTH_UNIT()
NAMED_UNIT(*)
SI_UNIT(.MILLI.,.METRE.)
) ;
#196744=(
NAMED_UNIT(*)
PLANE_ANGLE_UNIT()
SI_UNIT($,.RADIAN.)
) ;
#196745=(
NAMED_UNIT(*)
SI_UNIT($,.STERADIAN.)
SOLID_ANGLE_UNIT()
) ;
#196753=PRODUCT_DEFINITION_CONTEXT('part definition',#196761,'design') ;
#196761=APPLICATION_CONTEXT(
'Core Data for Automotive Mechanical Design Process') ;
#196762=PRODUCT_CONTEXT('part definition',#196761,'mechanical') ;
#196765=PRESENTATION_STYLE_ASSIGNMENT((#196767)) ;
#196767=SURFACE_STYLE_USAGE(.BOTH.,#196769) ;
#196769=SURFACE_SIDE_STYLE('',(#196771)) ;
#196771=SURFACE_STYLE_FILL_AREA(#196773) ;
#196773=FILL_AREA_STYLE('Steel - Satin',(#196775)) ;
#196775=FILL_AREA_STYLE_COLOUR('Steel - Satin',#196777) ;
#196777=COLOUR_RGB('Steel - Satin', 0.09019608, 0.27058824, 0.51372549) ;
#196995=CARTESIAN_POINT ( '', ( 0.0, 0.0, 0.0 ) ) ;
#196996=DIRECTION ( '', ( 0.0, 0.0, 1.0 ) ) ;
#196997=DIRECTION ( '', ( 1.0, 0.0, 0.0 ) ) ;
#196998=AXIS2_PLACEMENT_3D ( '', #196995, #196996, #196997 ) ;
#196999=ADVANCED_BREP_SHAPE_REPRESENTATION ( 'Composer Arm', ( #347, #196998, #197009, #197355 ), #196740 ) ;
#197000=PRODUCT( 'Composer Arm', 'Composer Arm', '', ( #196762 ) ) ;
#197001=PRODUCT_DEFINITION_FORMATION ( '', '', #197000 ) ;
#197002=PRODUCT_DEFINITION( 'Composer Arm', 'Composer Arm', #197001, #196753 ) ;
#197003=PRODUCT_DEFINITION_SHAPE ( '', '', #197002 ) ;
#197004=SHAPE_DEFINITION_REPRESENTATION ( #197003, #196999 ) ;
#197006=CARTESIAN_POINT ( '', ( 0.0, 0.0, 0.0 ) ) ;
#197007=DIRECTION ( '', ( 0.0, 0.0, 1.0 ) ) ;
#197008=DIRECTION ( '', ( 1.0, 0.0, 0.0 ) ) ;
#197009=AXIS2_PLACEMENT_3D ( '', #197006, #197007, #197008 ) ;
#197352=CARTESIAN_POINT ( '', ( 0.0, 0.0, 0.0 ) ) ;
#197353=DIRECTION ( '', ( 0.0, 0.0, 1.0 ) ) ;
#197354=DIRECTION ( '', ( 1.0, 0.0, 0.0 ) ) ;
#197355=AXIS2_PLACEMENT_3D ( '', #197352, #197353, #197354 ) ;
ENDSEC;
END-ISO-10303-21;
